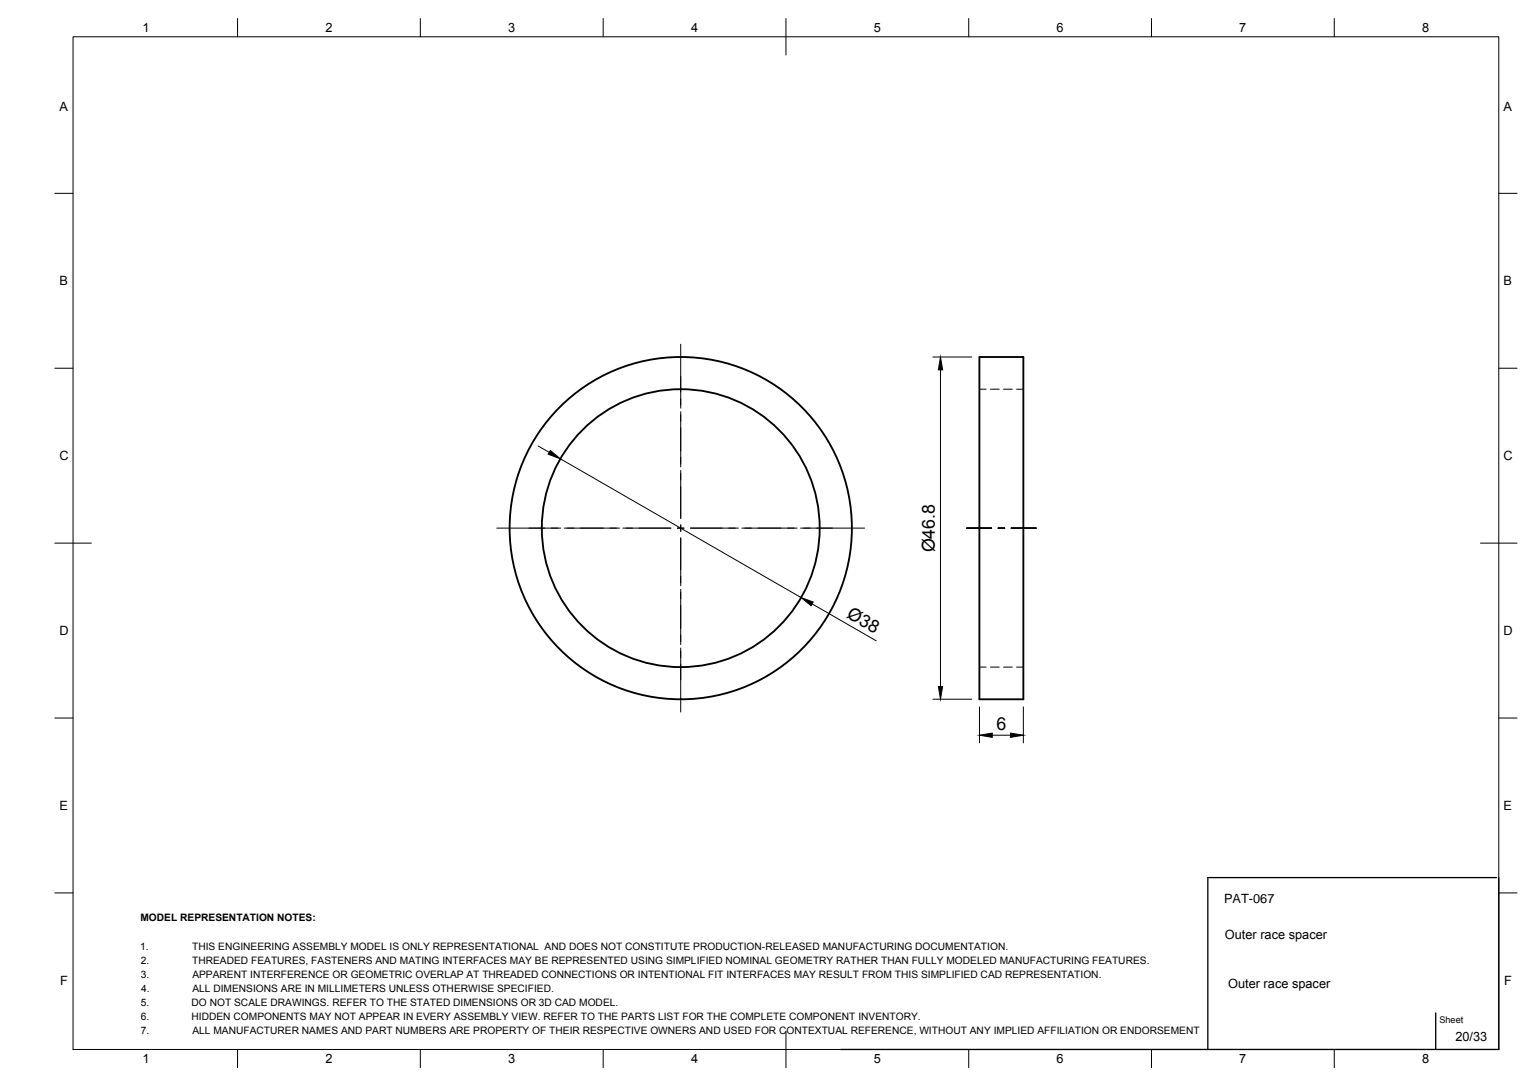
ISO-10303-21;
HEADER;
/* Generated by software containing ST-Developer
 * from STEP Tools, Inc. (www.steptools.com) 
 */

FILE_DESCRIPTION(
/* description */ ('Lifting hook block with sheave'),
/* implementation_level */ '2;1');

FILE_NAME(
/* name */ 'Outer race spacer.step',
/* time_stamp */ '2026-10-28T03:23:54-07:00',
/* author */ (''),
/* organization */ (''),
/* preprocessor_version */ 'ST-DEVELOPER v20.2',
/* originating_system */ 'Autodesk Translation Framework v15.17.0.0',
/* authorisation */ '');

FILE_SCHEMA (('AUTOMOTIVE_DESIGN { 1 0 10303 214 3 1 1 }'));
ENDSEC;

DATA;
#10=MECHANICAL_DESIGN_GEOMETRIC_PRESENTATION_REPRESENTATION('',(#368),#9391);
#308=SHAPE_REPRESENTATION_RELATIONSHIP('SRR','None',#9540,#338);
#338=ADVANCED_BREP_SHAPE_REPRESENTATION('',(#404),#9375);
#368=STYLED_ITEM('',(#9759),#404);
#404=MANIFOLD_SOLID_BREP('Body1',#4906);
#610=LINE('',#8380,#898);
#611=LINE('',#8386,#899);
#898=VECTOR('',#6849,1.9);
#899=VECTOR('',#6856,2.34);
#1065=CYLINDRICAL_SURFACE('',#5624,1.9);
#1066=CYLINDRICAL_SURFACE('',#5627,2.34);
#1178=FACE_BOUND('',#1748,.T.);
#1179=FACE_BOUND('',#1750,.T.);
#1385=FACE_OUTER_BOUND('',#1745,.T.);
#1386=FACE_OUTER_BOUND('',#1746,.T.);
#1387=FACE_OUTER_BOUND('',#1747,.T.);
#1388=FACE_OUTER_BOUND('',#1749,.T.);
#1745=EDGE_LOOP('',(#3938,#3939,#3940,#3941));
#1746=EDGE_LOOP('',(#3942,#3943,#3944,#3945));
#1747=EDGE_LOOP('',(#3946));
#1748=EDGE_LOOP('',(#3947));
#1749=EDGE_LOOP('',(#3948));
#1750=EDGE_LOOP('',(#3949));
#2071=CIRCLE('',#5625,1.9);
#2072=CIRCLE('',#5626,1.9);
#2073=CIRCLE('',#5628,2.34);
#2074=CIRCLE('',#5629,2.34);
#2440=VERTEX_POINT('',#8377);
#2441=VERTEX_POINT('',#8379);
#2442=VERTEX_POINT('',#8383);
#2443=VERTEX_POINT('',#8385);
#2973=EDGE_CURVE('',#2440,#2440,#2071,.T.);
#2974=EDGE_CURVE('',#2440,#2441,#610,.T.);
#2975=EDGE_CURVE('',#2441,#2441,#2072,.T.);
#2976=EDGE_CURVE('',#2442,#2442,#2073,.T.);
#2977=EDGE_CURVE('',#2442,#2443,#611,.T.);
#2978=EDGE_CURVE('',#2443,#2443,#2074,.T.);
#3938=ORIENTED_EDGE('',*,*,#2973,.F.);
#3939=ORIENTED_EDGE('',*,*,#2974,.T.);
#3940=ORIENTED_EDGE('',*,*,#2975,.T.);
#3941=ORIENTED_EDGE('',*,*,#2974,.F.);
#3942=ORIENTED_EDGE('',*,*,#2976,.F.);
#3943=ORIENTED_EDGE('',*,*,#2977,.T.);
#3944=ORIENTED_EDGE('',*,*,#2978,.T.);
#3945=ORIENTED_EDGE('',*,*,#2977,.F.);
#3946=ORIENTED_EDGE('',*,*,#2976,.T.);
#3947=ORIENTED_EDGE('',*,*,#2973,.T.);
#3948=ORIENTED_EDGE('',*,*,#2978,.F.);
#3949=ORIENTED_EDGE('',*,*,#2975,.F.);
#4539=PLANE('',#5630);
#4540=PLANE('',#5631);
#4761=ADVANCED_FACE('',(#1385),#1065,.F.);
#4762=ADVANCED_FACE('',(#1386),#1066,.T.);
#4763=ADVANCED_FACE('',(#1387,#1178),#4539,.T.);
#4764=ADVANCED_FACE('',(#1388,#1179),#4540,.F.);
#4906=CLOSED_SHELL('',(#4761,#4762,#4763,#4764));
#5623=AXIS2_PLACEMENT_3D('',#8375,#6843,#6844);
#5624=AXIS2_PLACEMENT_3D('',#8376,#6845,#6846);
#5625=AXIS2_PLACEMENT_3D('',#8378,#6847,#6848);
#5626=AXIS2_PLACEMENT_3D('',#8381,#6850,#6851);
#5627=AXIS2_PLACEMENT_3D('',#8382,#6852,#6853);
#5628=AXIS2_PLACEMENT_3D('',#8384,#6854,#6855);
#5629=AXIS2_PLACEMENT_3D('',#8387,#6857,#6858);
#5630=AXIS2_PLACEMENT_3D('',#8388,#6859,#6860);
#5631=AXIS2_PLACEMENT_3D('',#8389,#6861,#6862);
#6843=DIRECTION('axis',(0.,0.,1.));
#6844=DIRECTION('refdir',(1.,0.,0.));
#6845=DIRECTION('center_axis',(0.,1.,0.));
#6846=DIRECTION('ref_axis',(1.,0.,0.));
#6847=DIRECTION('center_axis',(0.,-1.,0.));
#6848=DIRECTION('ref_axis',(1.,0.,0.));
#6849=DIRECTION('',(0.,-1.,0.));
#6850=DIRECTION('center_axis',(0.,-1.,0.));
#6851=DIRECTION('ref_axis',(1.,0.,0.));
#6852=DIRECTION('center_axis',(0.,1.,0.));
#6853=DIRECTION('ref_axis',(1.,0.,0.));
#6854=DIRECTION('center_axis',(0.,1.,0.));
#6855=DIRECTION('ref_axis',(1.,0.,0.));
#6856=DIRECTION('',(0.,-1.,0.));
#6857=DIRECTION('center_axis',(0.,1.,0.));
#6858=DIRECTION('ref_axis',(1.,0.,0.));
#6859=DIRECTION('center_axis',(0.,1.,0.));
#6860=DIRECTION('ref_axis',(1.,0.,0.));
#6861=DIRECTION('center_axis',(0.,1.,0.));
#6862=DIRECTION('ref_axis',(1.,0.,0.));
#8375=CARTESIAN_POINT('',(0.,0.,0.));
#8376=CARTESIAN_POINT('Origin',(0.,-0.3,12.));
#8377=CARTESIAN_POINT('',(-1.9,0.3,12.));
#8378=CARTESIAN_POINT('Origin',(0.,0.3,12.));
#8379=CARTESIAN_POINT('',(-1.9,-0.3,12.));
#8380=CARTESIAN_POINT('',(-1.9,-0.3,12.));
#8381=CARTESIAN_POINT('Origin',(0.,-0.3,12.));
#8382=CARTESIAN_POINT('Origin',(0.,-0.3,12.));
#8383=CARTESIAN_POINT('',(-2.34,0.3,12.));
#8384=CARTESIAN_POINT('Origin',(0.,0.3,12.));
#8385=CARTESIAN_POINT('',(-2.34,-0.3,12.));
#8386=CARTESIAN_POINT('',(-2.34,-0.3,12.));
#8387=CARTESIAN_POINT('Origin',(0.,-0.3,12.));
#8388=CARTESIAN_POINT('Origin',(0.,0.3,12.));
#8389=CARTESIAN_POINT('Origin',(0.,-0.3,12.));
#9338=UNCERTAINTY_MEASURE_WITH_UNIT(LENGTH_MEASURE(0.001),#9392,
'DISTANCE_ACCURACY_VALUE',
'Maximum model space distance between geometric entities at asserted c
onnectivities');
#9354=UNCERTAINTY_MEASURE_WITH_UNIT(LENGTH_MEASURE(0.001),#9392,
'DISTANCE_ACCURACY_VALUE',
'Maximum model space distance between geometric entities at asserted c
onnectivities');
#9375=(
GEOMETRIC_REPRESENTATION_CONTEXT(3)
GLOBAL_UNCERTAINTY_ASSIGNED_CONTEXT((#9338))
GLOBAL_UNIT_ASSIGNED_CONTEXT((#9392,#9394,#9395))
REPRESENTATION_CONTEXT('','3D')
);
#9391=(
GEOMETRIC_REPRESENTATION_CONTEXT(3)
GLOBAL_UNCERTAINTY_ASSIGNED_CONTEXT((#9354))
GLOBAL_UNIT_ASSIGNED_CONTEXT((#9392,#9394,#9395))
REPRESENTATION_CONTEXT('','3D')
);
#9392=(
LENGTH_UNIT()
NAMED_UNIT(*)
SI_UNIT(.CENTI.,.METRE.)
);
#9394=(
NAMED_UNIT(*)
PLANE_ANGLE_UNIT()
SI_UNIT($,.RADIAN.)
);
#9395=(
NAMED_UNIT(*)
SI_UNIT($,.STERADIAN.)
SOLID_ANGLE_UNIT()
);
#9416=SHAPE_DEFINITION_REPRESENTATION(#9477,#9540);
#9477=PRODUCT_DEFINITION_SHAPE('',$,#9577);
#9540=SHAPE_REPRESENTATION('',(#5623),#9375);
#9556=PRODUCT_DEFINITION_CONTEXT('part definition',#9666,'design');
#9577=PRODUCT_DEFINITION('Outer race spacer','Outer race spacer',#9613,
#9556);
#9613=PRODUCT_DEFINITION_FORMATION('',$,#9688);
#9666=APPLICATION_CONTEXT(
'Core Data for Automotive Mechanical Design Process');
#9667=PRODUCT_CONTEXT('part definition',#9666,'mechanical');
#9688=PRODUCT('Outer race spacer','Outer race spacer',
'Outer race spacer',(#9667));
#9753=COLOUR_RGB('Grey',0.48,0.52,0.57);
#9754=FILL_AREA_STYLE_COLOUR('',#9753);
#9755=FILL_AREA_STYLE('',(#9754));
#9756=SURFACE_STYLE_FILL_AREA(#9755);
#9757=SURFACE_SIDE_STYLE('',(#9756));
#9758=SURFACE_STYLE_USAGE(.BOTH.,#9757);
#9759=PRESENTATION_STYLE_ASSIGNMENT((#9758));
ENDSEC;
END-ISO-10303-21;
